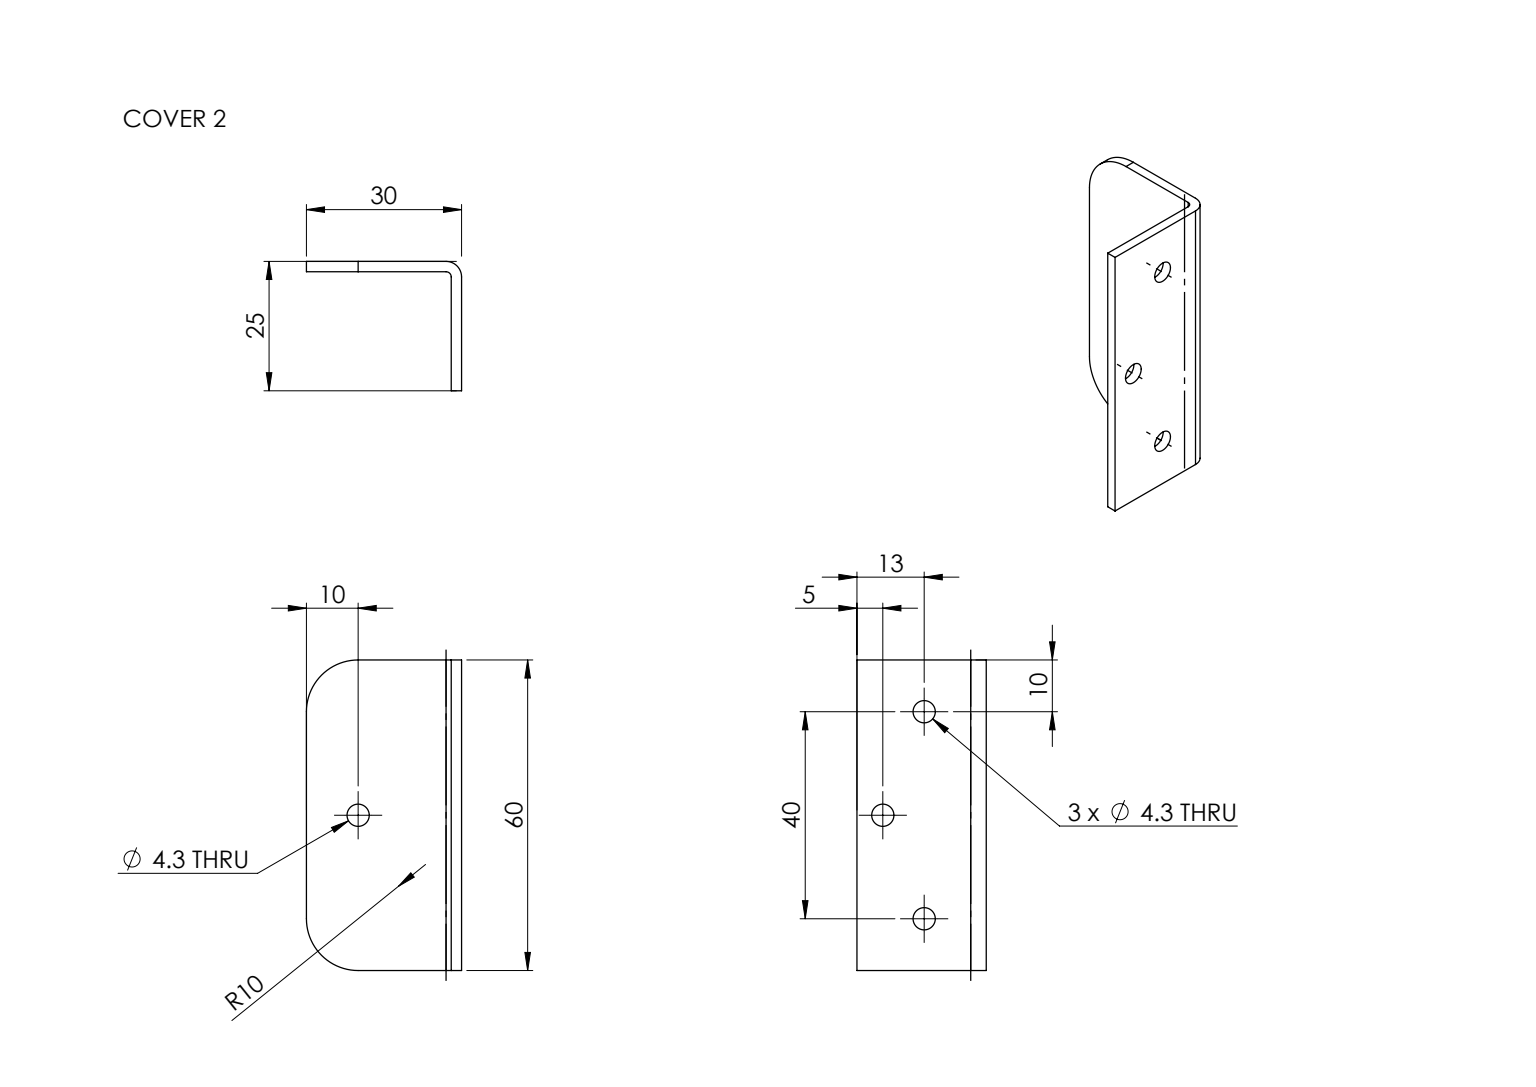
ISO-10303-21;
HEADER;
FILE_DESCRIPTION (('STEP AP214'),
    '1' );
FILE_NAME ('cover 2.step',
    '2026-10-03T20:08:58',
    ( '' ),
    ( '' ),
    'SwSTEP 2.0',
    'SolidWorks 2026',
    '' );
FILE_SCHEMA (( 'AUTOMOTIVE_DESIGN' ));
ENDSEC;

DATA;
#17=DIRECTION ( 'NONE',  ( 0.000000000000000000, 0.000000000000000000, 1.000000000000000000 ) ) ;
#30=LINE ( 'NONE', #10838, #312 ) ;
#47=VERTEX_POINT ( 'NONE', #5047 ) ;
#55=ORIENTED_EDGE ( 'NONE', *, *, #6653, .F. ) ;
#61=VECTOR ( 'NONE', #3554, 1000.000000000000000 ) ;
#80=CARTESIAN_POINT ( 'NONE',  ( -16.99999999999999289, 30.00000000000000000, 25.00000000000007105 ) ) ;
#104=FACE_OUTER_BOUND ( 'NONE', #9795, .T. ) ;
#120=EDGE_CURVE ( 'NONE', #10609, #7454, #4588, .T. ) ;
#131=DIRECTION ( 'NONE',  ( 0.000000000000000000, -1.177425296209236209E-30, -1.000000000000000000 ) ) ;
#140=CIRCLE ( 'NONE', #5087, 10.00000000000002309 ) ;
#209=COLOUR_RGB ( '', 0.66274510, 0.83137255, 0.94901961) ;
#213=EDGE_CURVE ( 'NONE', #4292, #815, #7867, .T. ) ;
#240=DIRECTION ( 'NONE',  ( -4.930380657631325535E-31, -1.000000000000000000, -1.177425296209239362E-30 ) ) ;
#259=CARTESIAN_POINT ( 'NONE',  ( -18.00000000000000355, 29.99999999999998224, 3.000000000000008438 ) ) ;
#261=CARTESIAN_POINT ( 'NONE',  ( -35.00000000000006395, 30.00000000000000000, 2.000000000000006661 ) ) ;
#263=CARTESIAN_POINT ( 'NONE',  ( -15.00000000000003375, 19.99999999999998934, 12.00000000000002842 ) ) ;
#279=CARTESIAN_POINT ( 'NONE',  ( -18.00000000000000355, 29.99999999999998224, 3.000000000000008438 ) ) ;
#280=( LENGTH_UNIT ( ) NAMED_UNIT ( * ) SI_UNIT ( .MILLI., .METRE. ) );
#302=VERTEX_POINT ( 'NONE', #12517 ) ;
#312=VECTOR ( 'NONE', #2087, 1000.000000000000000 ) ;
#352=CIRCLE ( 'NONE', #6535, 2.149999999999994138 ) ;
#364=VERTEX_POINT ( 'NONE', #10563 ) ;
#369=DIRECTION ( 'NONE',  ( 1.000000000000000000, 5.916456789157575403E-31, -1.577021341797098793E-16 ) ) ;
#455=CARTESIAN_POINT ( 'NONE',  ( -45.00000000000012079, -19.99999999999999645, 2.000000000000007994 ) ) ;
#471=DIRECTION ( 'NONE',  ( 0.000000000000000000, 0.000000000000000000, -1.000000000000000000 ) ) ;
#472=CARTESIAN_POINT ( 'NONE',  ( -17.00000000000000000, -30.00000000000000000, 3.000000000000030198 ) ) ;
#501=LINE ( 'NONE', #5270, #9745 ) ;
#507=EDGE_CURVE ( 'NONE', #8913, #7082, #5814, .T. ) ;
#509=VERTEX_POINT ( 'NONE', #8950 ) ;
#522=CARTESIAN_POINT ( 'NONE',  ( -18.00000000000002842, -30.00000000000000000, 4.336808689942017736E-16 ) ) ;
#538=CARTESIAN_POINT ( 'NONE',  ( -15.00000000000000000, 3.123110065765668157E-30, 22.15000000000006608 ) ) ;
#546=ORIENTED_EDGE ( 'NONE', *, *, #11077, .T. ) ;
#548=CARTESIAN_POINT ( 'NONE',  ( -15.00000000000003375, 19.99999999999998934, 12.00000000000002842 ) ) ;
#565=ORIENTED_EDGE ( 'NONE', *, *, #1103, .T. ) ;
#582=ORIENTED_EDGE ( 'NONE', *, *, #11922, .T. ) ;
#606=ADVANCED_FACE ( 'NONE', ( #5163 ), #9078, .F. ) ;
#609=DIRECTION ( 'NONE',  ( 1.000000000000000000, 5.916456789157575403E-31, -1.577021341797098793E-16 ) ) ;
#652=DIRECTION ( 'NONE',  ( -1.000000000000000000, -5.916456789157575403E-31, 1.577021341797098793E-16 ) ) ;
#681=LINE ( 'NONE', #4618, #8814 ) ;
#697=EDGE_LOOP ( 'NONE', ( #7888, #5340, #1354, #8282 ) ) ;
#703=CIRCLE ( 'NONE', #10980, 3.000000000000005773 ) ;
#708=EDGE_LOOP ( 'NONE', ( #5484, #4858 ) ) ;
#715=EDGE_CURVE ( 'NONE', #3334, #12136, #930, .T. ) ;
#724=PRODUCT ( 'cover 2', 'cover 2', '', ( #8914 ) ) ;
#734=DIRECTION ( 'NONE',  ( 1.000000000000000000, 5.916456789157575403E-31, -1.577021341797098793E-16 ) ) ;
#738=EDGE_LOOP ( 'NONE', ( #5945, #4675, #6555, #11845 ) ) ;
#749=VECTOR ( 'NONE', #6801, 1000.000000000000000 ) ;
#766=ADVANCED_FACE ( 'NONE', ( #4512, #5069, #893, #8688 ), #2728, .F. ) ;
#782=CARTESIAN_POINT ( 'NONE',  ( -35.00000000000006395, 19.99999999999999645, 2.000000000000006661 ) ) ;
#793=DIRECTION ( 'NONE',  ( 0.000000000000000000, 1.177425296209237785E-30, 1.000000000000000000 ) ) ;
#799=VECTOR ( 'NONE', #9430, 1000.000000000000000 ) ;
#808=AXIS2_PLACEMENT_3D ( 'NONE', #2794, #5790, #11854 ) ;
#813=DIRECTION ( 'NONE',  ( -1.000000000000000000, -5.916456789157575403E-31, 1.577021341797099039E-16 ) ) ;
#815=VERTEX_POINT ( 'NONE', #5661 ) ;
#822=ORIENTED_EDGE ( 'NONE', *, *, #9458, .T. ) ;
#834=CYLINDRICAL_SURFACE ( 'NONE', #10265, 2.149999999999999023 ) ;
#835=ORIENTED_EDGE ( 'NONE', *, *, #1795, .F. ) ;
#863=DIRECTION ( 'NONE',  ( -1.000000000000000000, -5.916456789157575403E-31, 1.577021341797098793E-16 ) ) ;
#884=AXIS2_PLACEMENT_3D ( 'NONE', #10014, #5142, #9121 ) ;
#893=FACE_BOUND ( 'NONE', #708, .T. ) ;
#926=DIRECTION ( 'NONE',  ( -1.000000000000000000, -5.916456789157575403E-31, 1.577021341797098793E-16 ) ) ;
#930=CIRCLE ( 'NONE', #7918, 10.00000000000002309 ) ;
#931=DIRECTION ( 'NONE',  ( 0.000000000000000000, 0.000000000000000000, -1.000000000000000000 ) ) ;
#954=LINE ( 'NONE', #3738, #5356 ) ;
#1019=CIRCLE ( 'NONE', #808, 2.149999999999994138 ) ;
#1060=DIRECTION ( 'NONE',  ( 1.000000000000000000, 5.916456789157575403E-31, -1.224646799147352714E-16 ) ) ;
#1071=ORIENTED_EDGE ( 'NONE', *, *, #6349, .F. ) ;
#1103=EDGE_CURVE ( 'NONE', #8313, #4963, #12522, .T. ) ;
#1114=EDGE_CURVE ( 'NONE', #11498, #6729, #11901, .T. ) ;
#1118=CYLINDRICAL_SURFACE ( 'NONE', #4514, 2.149999999999999023 ) ;
#1146=ORIENTED_EDGE ( 'NONE', *, *, #9111, .F. ) ;
#1156=DIRECTION ( 'NONE',  ( -4.930380657631325535E-31, -1.000000000000000000, -1.177425296209239362E-30 ) ) ;
#1166=DIRECTION ( 'NONE',  ( 0.000000000000000000, 0.000000000000000000, -1.000000000000000000 ) ) ;
#1176=DIRECTION ( 'NONE',  ( -4.930380657631325535E-31, -1.000000000000000000, -1.177425296209239362E-30 ) ) ;
#1179=AXIS2_PLACEMENT_3D ( 'NONE', #8679, #6694, #7716 ) ;
#1181=CARTESIAN_POINT ( 'NONE',  ( -18.00000000000001421, -30.00000000000001421, 3.000000000000008438 ) ) ;
#1199=ORIENTED_EDGE ( 'NONE', *, *, #5324, .F. ) ;
#1201=CARTESIAN_POINT ( 'NONE',  ( -18.00000000000002842, 30.00000000000000000, 4.336808689942017736E-16 ) ) ;
#1286=CARTESIAN_POINT ( 'NONE',  ( -15.00000000000000000, 2.465190328815661892E-29, 20.00000000000007461 ) ) ;
#1296=ADVANCED_FACE ( 'NONE', ( #7818 ), #3952, .T. ) ;
#1310=ORIENTED_EDGE ( 'NONE', *, *, #10574, .T. ) ;
#1318=ADVANCED_FACE ( 'NONE', ( #3131 ), #9024, .T. ) ;
#1354=ORIENTED_EDGE ( 'NONE', *, *, #5714, .F. ) ;
#1398=EDGE_CURVE ( 'NONE', #302, #815, #12426, .T. ) ;
#1402=DIRECTION ( 'NONE',  ( 1.000000000000000000, 5.916456789157575403E-31, -1.224646799147352714E-16 ) ) ;
#1452=CARTESIAN_POINT ( 'NONE',  ( -17.00000000000000000, 0.000000000000000000, 20.00000000000007461 ) ) ;
#1509=CARTESIAN_POINT ( 'NONE',  ( -45.00000000000001421, 19.99999999999999645, 3.443468848353431668E-15 ) ) ;
#1511=DIRECTION ( 'NONE',  ( -1.224646799147352714E-16, -1.177425296209236909E-30, -1.000000000000000000 ) ) ;
#1553=EDGE_CURVE ( 'NONE', #11498, #10609, #5066, .T. ) ;
#1561=CARTESIAN_POINT ( 'NONE',  ( -15.00000000000000711, -30.00000000000000000, 25.00000000000007105 ) ) ;
#1577=VERTEX_POINT ( 'NONE', #1907 ) ;
#1639=AXIS2_PLACEMENT_3D ( 'NONE', #5607, #12637, #7605 ) ;
#1662=CARTESIAN_POINT ( 'NONE',  ( -14.99999999999999289, 30.00000000000000000, 25.00000000000007105 ) ) ;
#1693=CARTESIAN_POINT ( 'NONE',  ( -15.00000000000000000, -20.00000000000000000, 14.15000000000002167 ) ) ;
#1702=CARTESIAN_POINT ( 'NONE',  ( -17.00000000000000000, 0.000000000000000000, 20.00000000000007461 ) ) ;
#1708=EDGE_CURVE ( 'NONE', #3334, #9611, #3336, .T. ) ;
#1734=VERTEX_POINT ( 'NONE', #11518 ) ;
#1766=DIRECTION ( 'NONE',  ( -1.000000000000000000, -5.916456789157575403E-31, 1.577021341797098793E-16 ) ) ;
#1779=( LENGTH_UNIT ( ) NAMED_UNIT ( * ) SI_UNIT ( .MILLI., .METRE. ) );
#1795=EDGE_CURVE ( 'NONE', #1734, #9663, #11530, .T. ) ;
#1850=AXIS2_PLACEMENT_3D ( 'NONE', #8562, #5785, #9765 ) ;
#1854=VECTOR ( 'NONE', #6775, 1000.000000000000000 ) ;
#1864=EDGE_CURVE ( 'NONE', #9310, #4937, #7061, .T. ) ;
#1886=ORIENTED_EDGE ( 'NONE', *, *, #6349, .T. ) ;
#1907=CARTESIAN_POINT ( 'NONE',  ( -15.00000000000003375, -30.00000000000000000, 3.000000000000029754 ) ) ;
#1922=ORIENTED_EDGE ( 'NONE', *, *, #7577, .F. ) ;
#1932=AXIS2_PLACEMENT_3D ( 'NONE', #2950, #3012, #4989 ) ;
#1936=CARTESIAN_POINT ( 'NONE',  ( -35.00000000000006395, -19.99999999999999645, 2.168404344971008868E-15 ) ) ;
#1941=LINE ( 'NONE', #6914, #4924 ) ;
#1958=DIRECTION ( 'NONE',  ( 0.000000000000000000, 1.177425296209236909E-30, 1.000000000000000000 ) ) ;
#1962=LINE ( 'NONE', #3904, #12124 ) ;
#1967=CARTESIAN_POINT ( 'NONE',  ( -35.00000000000006395, -2.157041537713704155E-29, 2.000000000000003553 ) ) ;
#1978=AXIS2_PLACEMENT_3D ( 'NONE', #1452, #926, #10645 ) ;
#2019=PRESENTATION_STYLE_ASSIGNMENT (( #6077 ) ) ;
#2087=DIRECTION ( 'NONE',  ( -2.465190328815656418E-32, 1.177425296209236734E-30, 1.000000000000000000 ) ) ;
#2088=AXIS2_PLACEMENT_3D ( 'NONE', #1286, #5281, #131 ) ;
#2104=AXIS2_PLACEMENT_3D ( 'NONE', #10365, #4392, #10559 ) ;
#2129=AXIS2_PLACEMENT_3D ( 'NONE', #3401, #12344, #3645 ) ;
#2143=( NAMED_UNIT ( * ) PLANE_ANGLE_UNIT ( ) SI_UNIT ( $, .RADIAN. ) );
#2145=ORIENTED_EDGE ( 'NONE', *, *, #10412, .T. ) ;
#2166=ORIENTED_EDGE ( 'NONE', *, *, #7676, .T. ) ;
#2167=CARTESIAN_POINT ( 'NONE',  ( -45.00000000000013500, 30.00000000000000000, 3.443468848353505426E-15 ) ) ;
#2207=CARTESIAN_POINT ( 'NONE',  ( -17.00000000000002842, 19.99999999999998579, 12.00000000000003730 ) ) ;
#2222=CARTESIAN_POINT ( 'NONE',  ( -18.00000000000002842, 30.00000000000000000, 2.000000000000004441 ) ) ;
#2233=DIRECTION ( 'NONE',  ( -1.000000000000000000, -5.916456789157575403E-31, 1.577021341797099039E-16 ) ) ;
#2244=EDGE_CURVE ( 'NONE', #11848, #1577, #6964, .T. ) ;
#2249=DIRECTION ( 'NONE',  ( 0.000000000000000000, 0.000000000000000000, -1.000000000000000000 ) ) ;
#2262=ORIENTED_EDGE ( 'NONE', *, *, #1795, .T. ) ;
#2285=MECHANICAL_DESIGN_GEOMETRIC_PRESENTATION_REPRESENTATION('',(#5766),#6810);
#2395=DIRECTION ( 'NONE',  ( -1.000000000000000000, 0.000000000000000000, 1.224646799147352714E-16 ) ) ;
#2408=CIRCLE ( 'NONE', #3443, 2.149999999999992362 ) ;
#2415=CARTESIAN_POINT ( 'NONE',  ( -17.00000000000002842, -20.00000000000000000, 9.850000000000047606 ) ) ;
#2421=ORIENTED_EDGE ( 'NONE', *, *, #8953, .T. ) ;
#2427=DIRECTION ( 'NONE',  ( -2.465190328815656418E-32, 1.177425296209236734E-30, 1.000000000000000000 ) ) ;
#2430=FACE_OUTER_BOUND ( 'NONE', #4109, .T. ) ;
#2442=CARTESIAN_POINT ( 'NONE',  ( -17.00000000000000000, 30.00000000000000000, 3.000000000000030198 ) ) ;
#2445=EDGE_LOOP ( 'NONE', ( #8731, #6641 ) ) ;
#2454=CARTESIAN_POINT ( 'NONE',  ( -16.99999999999999289, 30.00000000000000000, 25.00000000000007105 ) ) ;
#2494=DIRECTION ( 'NONE',  ( 0.000000000000000000, 0.000000000000000000, -1.000000000000000000 ) ) ;
#2500=FACE_OUTER_BOUND ( 'NONE', #3910, .T. ) ;
#2529=AXIS2_PLACEMENT_3D ( 'NONE', #11550, #2735, #9709 ) ;
#2583=PLANE ( 'NONE',  #11157 ) ;
#2592=CARTESIAN_POINT ( 'NONE',  ( -35.00000000000006395, -30.00000000000000000, 2.000000000000006661 ) ) ;
#2595=CARTESIAN_POINT ( 'NONE',  ( -15.00000000000000000, 30.00000000000000000, 3.000000000000029754 ) ) ;
#2597=EDGE_CURVE ( 'NONE', #4963, #9663, #954, .T. ) ;
#2635=FACE_BOUND ( 'NONE', #2445, .T. ) ;
#2648=FACE_BOUND ( 'NONE', #5059, .T. ) ;
#2695=VECTOR ( 'NONE', #1060, 1000.000000000000000 ) ;
#2697=EDGE_LOOP ( 'NONE', ( #5939, #9544, #4992, #8421 ) ) ;
#2710=DIRECTION ( 'NONE',  ( 1.000000000000000000, 5.916456789157576279E-31, 0.000000000000000000 ) ) ;
#2728=PLANE ( 'NONE',  #1850 ) ;
#2735=DIRECTION ( 'NONE',  ( -1.224646799147352714E-16, -1.177425296209236909E-30, -1.000000000000000000 ) ) ;
#2794=CARTESIAN_POINT ( 'NONE',  ( -17.00000000000002842, -20.00000000000000000, 12.00000000000003730 ) ) ;
#2825=APPLICATION_CONTEXT ( 'automotive_design' ) ;
#2839=CIRCLE ( 'NONE', #11249, 2.149999999999999023 ) ;
#2845=PRODUCT_DEFINITION_FORMATION_WITH_SPECIFIED_SOURCE ( 'ANY', '', #724, .NOT_KNOWN. ) ;
#2868=LINE ( 'NONE', #7803, #5698 ) ;
#2882=EDGE_CURVE ( 'NONE', #7500, #4292, #10406, .T. ) ;
#2883=LINE ( 'NONE', #5885, #749 ) ;
#2894=ORIENTED_EDGE ( 'NONE', *, *, #12398, .T. ) ;
#2912=ORIENTED_EDGE ( 'NONE', *, *, #2597, .T. ) ;
#2915=ORIENTED_EDGE ( 'NONE', *, *, #2244, .T. ) ;
#2949=AXIS2_PLACEMENT_3D ( 'NONE', #7795, #1156, #8946 ) ;
#2950=CARTESIAN_POINT ( 'NONE',  ( -35.00000000000006395, 19.99999999999999645, 2.000000000000007994 ) ) ;
#2964=ORIENTED_EDGE ( 'NONE', *, *, #1708, .F. ) ;
#3011=CARTESIAN_POINT ( 'NONE',  ( -17.00000000000002842, 19.99999999999998579, 12.00000000000003730 ) ) ;
#3012=DIRECTION ( 'NONE',  ( -2.465190328815656418E-32, 1.177425296209236734E-30, 1.000000000000000000 ) ) ;
#3015=AXIS2_PLACEMENT_3D ( 'NONE', #2222, #10051, #10116 ) ;
#3058=DIRECTION ( 'NONE',  ( -4.930380657631325535E-31, -1.000000000000000000, -1.177425296209239362E-30 ) ) ;
#3068=ORIENTED_EDGE ( 'NONE', *, *, #4877, .T. ) ;
#3074=ORIENTED_EDGE ( 'NONE', *, *, #11077, .F. ) ;
#3090=VECTOR ( 'NONE', #5249, 1000.000000000000000 ) ;
#3091=EDGE_LOOP ( 'NONE', ( #11028, #9675, #7446, #2915 ) ) ;
#3131=FACE_OUTER_BOUND ( 'NONE', #3091, .T. ) ;
#3143=ORIENTED_EDGE ( 'NONE', *, *, #5646, .T. ) ;
#3145=EDGE_CURVE ( 'NONE', #7082, #509, #5966, .T. ) ;
#3157=ORIENTED_EDGE ( 'NONE', *, *, #2882, .T. ) ;
#3175=ORIENTED_EDGE ( 'NONE', *, *, #12697, .T. ) ;
#3183=EDGE_CURVE ( 'NONE', #8913, #47, #6026, .T. ) ;
#3198=CARTESIAN_POINT ( 'NONE',  ( -32.85000000000007248, -2.147580246367739864E-29, 1.905105283154350624E-15 ) ) ;
#3199=ORIENTED_EDGE ( 'NONE', *, *, #5959, .T. ) ;
#3200=VECTOR ( 'NONE', #11397, 1000.000000000000000 ) ;
#3206=( NAMED_UNIT ( * ) SI_UNIT ( $, .STERADIAN. ) SOLID_ANGLE_UNIT ( ) );
#3223=AXIS2_PLACEMENT_3D ( 'NONE', #1181, #9032, #931 ) ;
#3242=VERTEX_POINT ( 'NONE', #6339 ) ;
#3244=ORIENTED_EDGE ( 'NONE', *, *, #8545, .T. ) ;
#3252=FACE_BOUND ( 'NONE', #3650, .T. ) ;
#3267=CARTESIAN_POINT ( 'NONE',  ( -18.00000000000001421, 29.99999999999999289, 2.000000000000004885 ) ) ;
#3283=VECTOR ( 'NONE', #813, 1000.000000000000000 ) ;
#3334=VERTEX_POINT ( 'NONE', #1509 ) ;
#3336=LINE ( 'NONE', #2167, #3090 ) ;
#3338=FACE_OUTER_BOUND ( 'NONE', #738, .T. ) ;
#3362=ADVANCED_FACE ( 'NONE', ( #7378 ), #10319, .F. ) ;
#3401=CARTESIAN_POINT ( 'NONE',  ( -17.00000000000002842, -20.00000000000000000, 12.00000000000003730 ) ) ;
#3405=ORIENTED_EDGE ( 'NONE', *, *, #507, .F. ) ;
#3407=ADVANCED_FACE ( 'NONE', ( #3584 ), #5311, .F. ) ;
#3408=PLANE ( 'NONE',  #3510 ) ;
#3439=ORIENTED_EDGE ( 'NONE', *, *, #10966, .T. ) ;
#3443=AXIS2_PLACEMENT_3D ( 'NONE', #1702, #1766, #793 ) ;
#3510=AXIS2_PLACEMENT_3D ( 'NONE', #5318, #12165, #4355 ) ;
#3519=STYLED_ITEM ( 'NONE', ( #11091 ), #9701 ) ;
#3546=AXIS2_PLACEMENT_3D ( 'NONE', #259, #4191, #8110 ) ;
#3554=DIRECTION ( 'NONE',  ( 1.000000000000000000, 5.916456789157575403E-31, -1.224646799147352714E-16 ) ) ;
#3584=FACE_OUTER_BOUND ( 'NONE', #11187, .T. ) ;
#3645=DIRECTION ( 'NONE',  ( 0.000000000000000000, 0.000000000000000000, 1.000000000000000000 ) ) ;
#3650=EDGE_LOOP ( 'NONE', ( #10523, #4157 ) ) ;
#3653=EDGE_LOOP ( 'NONE', ( #11585, #10453, #10007, #3765, #5718, #6710 ) ) ;
#3694=VECTOR ( 'NONE', #11699, 1000.000000000000000 ) ;
#3699=CARTESIAN_POINT ( 'NONE',  ( -18.00000000000001421, -30.00000000000001421, 3.000000000000008438 ) ) ;
#3734=DIRECTION ( 'NONE',  ( 5.916456789157575403E-31, -1.000000000000000000, -1.177425296209239362E-30 ) ) ;
#3738=CARTESIAN_POINT ( 'NONE',  ( -32.85000000000006537, -2.029837716746816226E-29, 2.000000000000002220 ) ) ;
#3765=ORIENTED_EDGE ( 'NONE', *, *, #12715, .T. ) ;
#3773=EDGE_CURVE ( 'NONE', #6729, #7454, #11229, .T. ) ;
#3795=DIRECTION ( 'NONE',  ( -2.465190328815656418E-32, 1.177425296209236734E-30, 1.000000000000000000 ) ) ;
#3904=CARTESIAN_POINT ( 'NONE',  ( -45.00000000000001421, 19.99999999999999645, 3.469446951953614189E-15 ) ) ;
#3910=EDGE_LOOP ( 'NONE', ( #9964, #4431, #3439, #2166 ) ) ;
#3940=DIRECTION ( 'NONE',  ( -4.930380657631325535E-31, -1.000000000000000000, -1.177425296209239362E-30 ) ) ;
#3952=PLANE ( 'NONE',  #5930 ) ;
#3956=VECTOR ( 'NONE', #6375, 1000.000000000000000 ) ;
#3984=DIRECTION ( 'NONE',  ( -2.465190328815656418E-32, 1.177425296209236734E-30, 1.000000000000000000 ) ) ;
#4014=DIRECTION ( 'NONE',  ( 1.000000000000000000, 5.916456789157575403E-31, 2.465190328815656418E-32 ) ) ;
#4067=SURFACE_SIDE_STYLE ('',( #8119 ) ) ;
#4109=EDGE_LOOP ( 'NONE', ( #6272, #6518, #11240, #8208 ) ) ;
#4134=FILL_AREA_STYLE ('',( #7708 ) ) ;
#4141=CARTESIAN_POINT ( 'NONE',  ( -18.00000000000000355, 29.99999999999998224, 3.000000000000008438 ) ) ;
#4157=ORIENTED_EDGE ( 'NONE', *, *, #1103, .F. ) ;
#4191=DIRECTION ( 'NONE',  ( -4.930380657631325535E-31, -1.000000000000000000, -1.177425296209239362E-30 ) ) ;
#4213=ORIENTED_EDGE ( 'NONE', *, *, #7256, .T. ) ;
#4231=ORIENTED_EDGE ( 'NONE', *, *, #1553, .T. ) ;
#4250=VERTEX_POINT ( 'NONE', #1662 ) ;
#4262=AXIS2_PLACEMENT_3D ( 'NONE', #5297, #9980, #7244 ) ;
#4282=DIRECTION ( 'NONE',  ( -1.000000000000000000, -5.916456789157575403E-31, 1.577021341797099039E-16 ) ) ;
#4292=VERTEX_POINT ( 'NONE', #10660 ) ;
#4312=CARTESIAN_POINT ( 'NONE',  ( -17.00000000000000000, 30.00000000000000000, 3.000000000000030198 ) ) ;
#4319=ADVANCED_FACE ( 'NONE', ( #104 ), #6821, .T. ) ;
#4331=CARTESIAN_POINT ( 'NONE',  ( -17.00000000000002842, -20.00000000000000000, 9.850000000000036948 ) ) ;
#4349=CARTESIAN_POINT ( 'NONE',  ( -35.00000000000006395, -19.99999999999999645, 3.000000000000008438 ) ) ;
#4355=DIRECTION ( 'NONE',  ( -1.577021341797098546E-16, -1.177425296209237084E-30, -1.000000000000000000 ) ) ;
#4392=DIRECTION ( 'NONE',  ( -1.000000000000000000, -5.916456789157575403E-31, 1.577021341797098793E-16 ) ) ;
#4431=ORIENTED_EDGE ( 'NONE', *, *, #2244, .F. ) ;
#4469=VECTOR ( 'NONE', #8952, 1000.000000000000000 ) ;
#4512=FACE_OUTER_BOUND ( 'NONE', #697, .T. ) ;
#4514=AXIS2_PLACEMENT_3D ( 'NONE', #8971, #8004, #1958 ) ;
#4570=LINE ( 'NONE', #8548, #3200 ) ;
#4588=CIRCLE ( 'NONE', #10542, 2.149999999999994138 ) ;
#4607=ORIENTED_EDGE ( 'NONE', *, *, #7208, .F. ) ;
#4618=CARTESIAN_POINT ( 'NONE',  ( -15.00000000000000000, 30.00000000000000000, 3.000000000000029754 ) ) ;
#4675=ORIENTED_EDGE ( 'NONE', *, *, #7256, .F. ) ;
#4706=LINE ( 'NONE', #12578, #6378 ) ;
#4734=DIRECTION ( 'NONE',  ( 1.000000000000000000, 5.916456789157576279E-31, 0.000000000000000000 ) ) ;
#4740=ADVANCED_FACE ( 'NONE', ( #2430 ), #6342, .F. ) ;
#4746=ORIENTED_EDGE ( 'NONE', *, *, #5952, .F. ) ;
#4788=UNCERTAINTY_MEASURE_WITH_UNIT (LENGTH_MEASURE( 1.000000000000000082E-05 ), #10955, 'distance_accuracy_value', 'NONE');
#4796=CIRCLE ( 'NONE', #884, 10.00000000000002309 ) ;
#4804=AXIS2_PLACEMENT_3D ( 'NONE', #12219, #2427, #4854 ) ;
#4854=DIRECTION ( 'NONE',  ( 1.000000000000000000, 5.916456789157576279E-31, 0.000000000000000000 ) ) ;
#4858=ORIENTED_EDGE ( 'NONE', *, *, #11792, .F. ) ;
#4876=AXIS2_PLACEMENT_3D ( 'NONE', #4349, #9229, #8276 ) ;
#4877=EDGE_CURVE ( 'NONE', #3242, #9347, #2883, .T. ) ;
#4924=VECTOR ( 'NONE', #6972, 1000.000000000000000 ) ;
#4937=VERTEX_POINT ( 'NONE', #6073 ) ;
#4963=VERTEX_POINT ( 'NONE', #3198 ) ;
#4989=DIRECTION ( 'NONE',  ( 1.000000000000000000, 0.000000000000000000, 0.000000000000000000 ) ) ;
#4992=ORIENTED_EDGE ( 'NONE', *, *, #11792, .T. ) ;
#5043=( NAMED_UNIT ( * ) SI_UNIT ( $, .STERADIAN. ) SOLID_ANGLE_UNIT ( ) );
#5047=CARTESIAN_POINT ( 'NONE',  ( -17.00000000000000000, 2.531464386849852200E-30, 22.15000000000006608 ) ) ;
#5059=EDGE_LOOP ( 'NONE', ( #3405, #12376 ) ) ;
#5061=ORIENTED_EDGE ( 'NONE', *, *, #10966, .F. ) ;
#5066=LINE ( 'NONE', #11642, #3694 ) ;
#5069=FACE_BOUND ( 'NONE', #12624, .T. ) ;
#5087=AXIS2_PLACEMENT_3D ( 'NONE', #1936, #12520, #7616 ) ;
#5116=( NAMED_UNIT ( * ) PLANE_ANGLE_UNIT ( ) SI_UNIT ( $, .RADIAN. ) );
#5123=ORIENTED_EDGE ( 'NONE', *, *, #11983, .F. ) ;
#5128=CIRCLE ( 'NONE', #11295, 2.149999999999999023 ) ;
#5141=AXIS2_PLACEMENT_3D ( 'NONE', #1967, #10535, #2710 ) ;
#5142=DIRECTION ( 'NONE',  ( 1.224646799147352714E-16, 1.177425296209236909E-30, 1.000000000000000000 ) ) ;
#5163=FACE_OUTER_BOUND ( 'NONE', #8488, .T. ) ;
#5217=EDGE_LOOP ( 'NONE', ( #11701, #3199, #3068, #3244, #2421, #7025, #1199, #6196 ) ) ;
#5249=DIRECTION ( 'NONE',  ( -4.930380657631325535E-31, -1.000000000000000000, -1.177425296209239362E-30 ) ) ;
#5250=CARTESIAN_POINT ( 'NONE',  ( -17.00000000000000000, 2.531464386849858155E-30, 22.15000000000007319 ) ) ;
#5270=CARTESIAN_POINT ( 'NONE',  ( -18.00000000000002842, 30.00000000000000000, 2.000000000000004441 ) ) ;
#5276=ORIENTED_EDGE ( 'NONE', *, *, #3773, .T. ) ;
#5281=DIRECTION ( 'NONE',  ( 1.000000000000000000, 5.916456789157575403E-31, -1.577021341797098793E-16 ) ) ;
#5297=CARTESIAN_POINT ( 'NONE',  ( -17.00000000000002842, -20.00000000000000000, 12.00000000000003730 ) ) ;
#5301=EDGE_CURVE ( 'NONE', #3242, #9611, #140, .T. ) ;
#5311=CYLINDRICAL_SURFACE ( 'NONE', #4804, 2.149999999999999023 ) ;
#5318=CARTESIAN_POINT ( 'NONE',  ( -15.00000000000000000, 30.00000000000000000, 3.000000000000029754 ) ) ;
#5324=EDGE_CURVE ( 'NONE', #10180, #8458, #11806, .T. ) ;
#5340=ORIENTED_EDGE ( 'NONE', *, *, #12250, .F. ) ;
#5356=VECTOR ( 'NONE', #3984, 1000.000000000000000 ) ;
#5359=CARTESIAN_POINT ( 'NONE',  ( -17.00000000000002842, 19.99999999999998579, 12.00000000000003730 ) ) ;
#5397=DIRECTION ( 'NONE',  ( -2.465190328815656418E-32, 1.177425296209236734E-30, 1.000000000000000000 ) ) ;
#5399=CARTESIAN_POINT ( 'NONE',  ( -16.99999999999999289, -30.00000000000000000, 25.00000000000007105 ) ) ;
#5404=CARTESIAN_POINT ( 'NONE',  ( -35.00000000000006395, 30.00000000000000000, 2.218822049206179977E-15 ) ) ;
#5423=ORIENTED_EDGE ( 'NONE', *, *, #5431, .T. ) ;
#5431=EDGE_CURVE ( 'NONE', #815, #4292, #352, .T. ) ;
#5444=DIRECTION ( 'NONE',  ( 0.000000000000000000, 0.000000000000000000, -1.000000000000000000 ) ) ;
#5480=AXIS2_PLACEMENT_3D ( 'NONE', #10079, #369, #2249 ) ;
#5484=ORIENTED_EDGE ( 'NONE', *, *, #5909, .F. ) ;
#5526=EDGE_LOOP ( 'NONE', ( #11382, #5843, #1886, #12256 ) ) ;
#5531=CARTESIAN_POINT ( 'NONE',  ( -32.85000000000006537, -2.029837716746816226E-29, 2.000000000000003553 ) ) ;
#5535=DIRECTION ( 'NONE',  ( -1.000000000000000000, -5.916456789157575403E-31, -2.465190328815656418E-32 ) ) ;
#5583=ORIENTED_EDGE ( 'NONE', *, *, #9111, .T. ) ;
#5607=CARTESIAN_POINT ( 'NONE',  ( -15.00000000000000000, 2.465190328815661892E-29, 20.00000000000007461 ) ) ;
#5609=AXIS2_PLACEMENT_3D ( 'NONE', #5359, #652, #6592 ) ;
#5646=EDGE_CURVE ( 'NONE', #6729, #11498, #9769, .T. ) ;
#5661=CARTESIAN_POINT ( 'NONE',  ( -17.00000000000002842, 19.99999999999998579, 14.15000000000003055 ) ) ;
#5692=CARTESIAN_POINT ( 'NONE',  ( -35.00000000000006395, -2.157041537713704155E-29, 2.000000000000003553 ) ) ;
#5698=VECTOR ( 'NONE', #5927, 1000.000000000000000 ) ;
#5707=CARTESIAN_POINT ( 'NONE',  ( 0.000000000000000000, 0.000000000000000000, 0.000000000000000000 ) ) ;
#5713=ORIENTED_EDGE ( 'NONE', *, *, #8690, .F. ) ;
#5714=EDGE_CURVE ( 'NONE', #12227, #11665, #7395, .T. ) ;
#5718=ORIENTED_EDGE ( 'NONE', *, *, #1864, .T. ) ;
#5719=LINE ( 'NONE', #9630, #10320 ) ;
#5747=AXIS2_PLACEMENT_3D ( 'NONE', #3699, #11559, #11023 ) ;
#5750=AXIS2_PLACEMENT_3D ( 'NONE', #6673, #1511, #10584 ) ;
#5765=( GEOMETRIC_REPRESENTATION_CONTEXT ( 3 ) GLOBAL_UNCERTAINTY_ASSIGNED_CONTEXT ( ( #11494 ) ) GLOBAL_UNIT_ASSIGNED_CONTEXT ( ( #1779, #12482, #5043 ) ) REPRESENTATION_CONTEXT ( 'NONE', 'WORKASPACE' ) );
#5766=STYLED_ITEM ( 'NONE', ( #2019 ), #10029 ) ;
#5785=DIRECTION ( 'NONE',  ( 1.000000000000000000, 5.916456789157575403E-31, -1.577021341797098546E-16 ) ) ;
#5790=DIRECTION ( 'NONE',  ( -1.000000000000000000, -5.916456789157575403E-31, 1.577021341797098793E-16 ) ) ;
#5798=CIRCLE ( 'NONE', #2529, 2.149999999999999023 ) ;
#5805=CARTESIAN_POINT ( 'NONE',  ( -17.00000000000002842, 19.99999999999998579, 12.00000000000003730 ) ) ;
#5809=ADVANCED_FACE ( 'NONE', ( #3338 ), #10186, .T. ) ;
#5814=CIRCLE ( 'NONE', #2088, 2.149999999999999023 ) ;
#5828=ORIENTED_EDGE ( 'NONE', *, *, #1553, .F. ) ;
#5843=ORIENTED_EDGE ( 'NONE', *, *, #7676, .F. ) ;
#5885=CARTESIAN_POINT ( 'NONE',  ( -18.00000000000002842, -30.00000000000000000, 1.369224906555730040E-16 ) ) ;
#5909=EDGE_CURVE ( 'NONE', #47, #509, #2408, .T. ) ;
#5913=ORIENTED_EDGE ( 'NONE', *, *, #120, .F. ) ;
#5923=EDGE_CURVE ( 'NONE', #9663, #1734, #6930, .T. ) ;
#5927=DIRECTION ( 'NONE',  ( -1.000000000000000000, -5.916456789157575403E-31, -2.465190328815656418E-32 ) ) ;
#5930=AXIS2_PLACEMENT_3D ( 'NONE', #11816, #10832, #4014 ) ;
#5939=ORIENTED_EDGE ( 'NONE', *, *, #507, .T. ) ;
#5945=ORIENTED_EDGE ( 'NONE', *, *, #12715, .F. ) ;
#5946=DIRECTION ( 'NONE',  ( 0.000000000000000000, 0.000000000000000000, 1.000000000000000000 ) ) ;
#5952=EDGE_CURVE ( 'NONE', #302, #7500, #2839, .T. ) ;
#5959=EDGE_CURVE ( 'NONE', #9310, #3242, #6413, .T. ) ;
#5963=AXIS2_PLACEMENT_3D ( 'NONE', #8893, #3058, #6973 ) ;
#5966=LINE ( 'NONE', #7257, #9914 ) ;
#6018=ORIENTED_EDGE ( 'NONE', *, *, #120, .T. ) ;
#6026=LINE ( 'NONE', #5250, #12418 ) ;
#6062=DIRECTION ( 'NONE',  ( 1.000000000000000000, 5.916456789157575403E-31, -1.577021341797098793E-16 ) ) ;
#6073=CARTESIAN_POINT ( 'NONE',  ( -18.00000000000001421, -30.00000000000000711, 2.000000000000004885 ) ) ;
#6075=FACE_BOUND ( 'NONE', #6886, .T. ) ;
#6077=SURFACE_STYLE_USAGE ( .BOTH. , #8065 ) ;
#6086=ADVANCED_FACE ( 'NONE', ( #8261 ), #11162, .F. ) ;
#6102=LINE ( 'NONE', #1201, #11999 ) ;
#6112=VECTOR ( 'NONE', #8579, 1000.000000000000000 ) ;
#6125=DIRECTION ( 'NONE',  ( -1.000000000000000000, -5.916456789157575403E-31, 1.577021341797098793E-16 ) ) ;
#6133=CARTESIAN_POINT ( 'NONE',  ( -17.00000000000002842, -20.00000000000000000, 12.00000000000003730 ) ) ;
#6135=AXIS2_PLACEMENT_3D ( 'NONE', #4141, #1176, #7046 ) ;
#6196=ORIENTED_EDGE ( 'NONE', *, *, #10412, .F. ) ;
#6239=EDGE_CURVE ( 'NONE', #8666, #8458, #10305, .T. ) ;
#6272=ORIENTED_EDGE ( 'NONE', *, *, #3145, .F. ) ;
#6290=ORIENTED_EDGE ( 'NONE', *, *, #715, .T. ) ;
#6316=DIRECTION ( 'NONE',  ( -1.000000000000000000, -5.916456789157575403E-31, 1.224646799147352714E-16 ) ) ;
#6339=CARTESIAN_POINT ( 'NONE',  ( -35.00000000000006395, -30.00000000000000000, 2.218822049206081369E-15 ) ) ;
#6342=CYLINDRICAL_SURFACE ( 'NONE', #1978, 2.149999999999999023 ) ;
#6349=EDGE_CURVE ( 'NONE', #4250, #11665, #2868, .T. ) ;
#6375=DIRECTION ( 'NONE',  ( -4.930380657631325535E-31, -1.000000000000000000, -1.177425296209239362E-30 ) ) ;
#6378=VECTOR ( 'NONE', #6519, 1000.000000000000000 ) ;
#6413=LINE ( 'NONE', #12662, #6525 ) ;
#6428=DIRECTION ( 'NONE',  ( 1.000000000000000000, 0.000000000000000000, 0.000000000000000000 ) ) ;
#6430=DIRECTION ( 'NONE',  ( 1.577021341797099039E-16, 1.177425296209237084E-30, 1.000000000000000000 ) ) ;
#6431=ORIENTED_EDGE ( 'NONE', *, *, #715, .F. ) ;
#6443=ORIENTED_EDGE ( 'NONE', *, *, #1398, .F. ) ;
#6507=ORIENTED_EDGE ( 'NONE', *, *, #5923, .F. ) ;
#6518=ORIENTED_EDGE ( 'NONE', *, *, #10714, .T. ) ;
#6519=DIRECTION ( 'NONE',  ( -4.930380657631325535E-31, -1.000000000000000000, -1.177425296209239362E-30 ) ) ;
#6525=VECTOR ( 'NONE', #7757, 1000.000000000000000 ) ;
#6529=EDGE_CURVE ( 'NONE', #7823, #8669, #501, .T. ) ;
#6533=DIRECTION ( 'NONE',  ( -1.000000000000000000, 0.000000000000000000, 1.301042606982602363E-16 ) ) ;
#6535=AXIS2_PLACEMENT_3D ( 'NONE', #2207, #6125, #10034 ) ;
#6538=FACE_OUTER_BOUND ( 'NONE', #5217, .T. ) ;
#6555=ORIENTED_EDGE ( 'NONE', *, *, #5301, .F. ) ;
#6560=ORIENTED_EDGE ( 'NONE', *, *, #6612, .T. ) ;
#6569=ORIENTED_EDGE ( 'NONE', *, *, #1398, .T. ) ;
#6592=DIRECTION ( 'NONE',  ( 0.000000000000000000, 0.000000000000000000, 1.000000000000000000 ) ) ;
#6612=EDGE_CURVE ( 'NONE', #12136, #7823, #11267, .T. ) ;
#6641=ORIENTED_EDGE ( 'NONE', *, *, #5646, .F. ) ;
#6653=EDGE_CURVE ( 'NONE', #12092, #7976, #4570, .T. ) ;
#6673=CARTESIAN_POINT ( 'NONE',  ( -35.00000000000006395, -2.157041537713704155E-29, 2.168404344971033323E-15 ) ) ;
#6694=DIRECTION ( 'NONE',  ( -1.000000000000000000, -5.916456789157575403E-31, -2.465190328815656418E-32 ) ) ;
#6710=ORIENTED_EDGE ( 'NONE', *, *, #10574, .F. ) ;
#6729=VERTEX_POINT ( 'NONE', #11587 ) ;
#6775=DIRECTION ( 'NONE',  ( -4.930380657631325535E-31, -1.000000000000000000, -1.177425296209239362E-30 ) ) ;
#6776=AXIS2_PLACEMENT_3D ( 'NONE', #11279, #11996, #6316 ) ;
#6784=CARTESIAN_POINT ( 'NONE',  ( -14.99999999999999289, 30.00000000000000000, 25.00000000000007105 ) ) ;
#6801=DIRECTION ( 'NONE',  ( 1.000000000000000000, 5.916456789157575403E-31, -1.224646799147352714E-16 ) ) ;
#6803=CARTESIAN_POINT ( 'NONE',  ( -17.00000000000000000, 30.00000000000000000, 3.000000000000030198 ) ) ;
#6809=EDGE_LOOP ( 'NONE', ( #2964, #6290, #11253, #3175, #8753, #10302 ) ) ;
#6810=( GEOMETRIC_REPRESENTATION_CONTEXT ( 3 ) GLOBAL_UNCERTAINTY_ASSIGNED_CONTEXT ( ( #8653 ) ) GLOBAL_UNIT_ASSIGNED_CONTEXT ( ( #280, #5116, #3206 ) ) REPRESENTATION_CONTEXT ( 'NONE', 'WORKASPACE' ) );
#6812=SURFACE_STYLE_USAGE ( .BOTH. , #4067 ) ;
#6821=PLANE ( 'NONE',  #1179 ) ;
#6874=SHAPE_DEFINITION_REPRESENTATION ( #8540, #11514 ) ;
#6886=EDGE_LOOP ( 'NONE', ( #6507, #835 ) ) ;
#6914=CARTESIAN_POINT ( 'NONE',  ( -15.00000000000003375, -30.00000000000000000, 3.000000000000029754 ) ) ;
#6927=DIRECTION ( 'NONE',  ( -4.930380657631325535E-31, -1.000000000000000000, -1.177425296209239362E-30 ) ) ;
#6930=CIRCLE ( 'NONE', #9576, 2.149999999999999023 ) ;
#6964=LINE ( 'NONE', #11923, #1854 ) ;
#6972=DIRECTION ( 'NONE',  ( 1.577021341797099039E-16, 1.177425296209237084E-30, 1.000000000000000000 ) ) ;
#6973=DIRECTION ( 'NONE',  ( 1.000000000000000000, 0.000000000000000000, -6.375108774214761023E-14 ) ) ;
#7025=ORIENTED_EDGE ( 'NONE', *, *, #6239, .T. ) ;
#7046=DIRECTION ( 'NONE',  ( 0.000000000000000000, 0.000000000000000000, -1.000000000000000000 ) ) ;
#7052=FILL_AREA_STYLE ('',( #11760 ) ) ;
#7061=LINE ( 'NONE', #10913, #2695 ) ;
#7082=VERTEX_POINT ( 'NONE', #12474 ) ;
#7106=ORIENTED_EDGE ( 'NONE', *, *, #213, .T. ) ;
#7117=VECTOR ( 'NONE', #3940, 1000.000000000000000 ) ;
#7118=ORIENTED_EDGE ( 'NONE', *, *, #2882, .F. ) ;
#7164=CARTESIAN_POINT ( 'NONE',  ( -17.00000000000000000, -30.00000000000000000, 3.000000000000030198 ) ) ;
#7208=EDGE_CURVE ( 'NONE', #12227, #10180, #12728, .T. ) ;
#7242=ADVANCED_FACE ( 'NONE', ( #8844 ), #7878, .F. ) ;
#7244=DIRECTION ( 'NONE',  ( 0.000000000000000000, 0.000000000000000000, 1.000000000000000000 ) ) ;
#7256=EDGE_CURVE ( 'NONE', #9611, #7976, #30, .T. ) ;
#7257=CARTESIAN_POINT ( 'NONE',  ( -17.00000000000000000, 2.632990618166788035E-16, 17.85000000000007248 ) ) ;
#7274=EDGE_LOOP ( 'NONE', ( #1922, #9378, #6431, #3074 ) ) ;
#7307=FACE_OUTER_BOUND ( 'NONE', #3653, .T. ) ;
#7340=ADVANCED_FACE ( 'NONE', ( #6075, #7307 ), #9281, .F. ) ;
#7346=ORIENTED_EDGE ( 'NONE', *, *, #5952, .T. ) ;
#7355=PLANE ( 'NONE',  #6776 ) ;
#7378=FACE_OUTER_BOUND ( 'NONE', #9057, .T. ) ;
#7392=DIRECTION ( 'NONE',  ( 0.000000000000000000, 0.000000000000000000, 1.000000000000000000 ) ) ;
#7395=LINE ( 'NONE', #2442, #12692 ) ;
#7407=AXIS2_PLACEMENT_3D ( 'NONE', #9411, #609, #5444 ) ;
#7446=ORIENTED_EDGE ( 'NONE', *, *, #8690, .T. ) ;
#7454=VERTEX_POINT ( 'NONE', #2415 ) ;
#7457=CARTESIAN_POINT ( 'NONE',  ( -17.00000000000002842, 19.99999999999998579, 14.15000000000003588 ) ) ;
#7500=VERTEX_POINT ( 'NONE', #8389 ) ;
#7510=AXIS2_PLACEMENT_3D ( 'NONE', #3011, #863, #5946 ) ;
#7577=EDGE_CURVE ( 'NONE', #7823, #12092, #12466, .T. ) ;
#7605=DIRECTION ( 'NONE',  ( 0.000000000000000000, -1.177425296209236209E-30, -1.000000000000000000 ) ) ;
#7616=DIRECTION ( 'NONE',  ( -1.000000000000000000, 0.000000000000000000, 1.224646799147352714E-16 ) ) ;
#7676=EDGE_CURVE ( 'NONE', #4250, #8666, #10633, .T. ) ;
#7703=DIRECTION ( 'NONE',  ( 2.465190328815656418E-32, -1.177425296209236734E-30, -1.000000000000000000 ) ) ;
#7704=EDGE_LOOP ( 'NONE', ( #7346, #3157, #7106, #6443 ) ) ;
#7708=FILL_AREA_STYLE_COLOUR ( '', #209 ) ;
#7716=DIRECTION ( 'NONE',  ( -2.465190328815656418E-32, 1.177425296209236734E-30, 1.000000000000000000 ) ) ;
#7757=DIRECTION ( 'NONE',  ( 2.465190328815656418E-32, -1.177425296209236734E-30, -1.000000000000000000 ) ) ;
#7795=CARTESIAN_POINT ( 'NONE',  ( -18.00000000000000355, 29.99999999999998224, 3.000000000000008438 ) ) ;
#7803=CARTESIAN_POINT ( 'NONE',  ( -14.99999999999999289, 30.00000000000000000, 25.00000000000007105 ) ) ;
#7818=FACE_OUTER_BOUND ( 'NONE', #5526, .T. ) ;
#7823=VERTEX_POINT ( 'NONE', #261 ) ;
#7825=FACE_OUTER_BOUND ( 'NONE', #7274, .T. ) ;
#7867=CIRCLE ( 'NONE', #5609, 2.149999999999994138 ) ;
#7878=CYLINDRICAL_SURFACE ( 'NONE', #7510, 2.149999999999999023 ) ;
#7888=ORIENTED_EDGE ( 'NONE', *, *, #5324, .T. ) ;
#7918=AXIS2_PLACEMENT_3D ( 'NONE', #8372, #12248, #2395 ) ;
#7976=VERTEX_POINT ( 'NONE', #455 ) ;
#8004=DIRECTION ( 'NONE',  ( -1.000000000000000000, -5.916456789157575403E-31, 1.577021341797098793E-16 ) ) ;
#8046=CIRCLE ( 'NONE', #2104, 2.149999999999992362 ) ;
#8065=SURFACE_SIDE_STYLE ('',( #10774 ) ) ;
#8105=LINE ( 'NONE', #2454, #3956 ) ;
#8110=DIRECTION ( 'NONE',  ( 0.000000000000000000, 0.000000000000000000, -1.000000000000000000 ) ) ;
#8119=SURFACE_STYLE_FILL_AREA ( #4134 ) ;
#8208=ORIENTED_EDGE ( 'NONE', *, *, #5909, .T. ) ;
#8260=DIRECTION ( 'NONE',  ( -1.000000000000000000, -5.916456789157575403E-31, 1.577021341797099039E-16 ) ) ;
#8261=FACE_OUTER_BOUND ( 'NONE', #12309, .T. ) ;
#8276=DIRECTION ( 'NONE',  ( -1.000000000000000000, 0.000000000000000000, 0.000000000000000000 ) ) ;
#8282=ORIENTED_EDGE ( 'NONE', *, *, #7208, .T. ) ;
#8291=CARTESIAN_POINT ( 'NONE',  ( -17.00000000000002842, 19.99999999999998579, 9.850000000000036948 ) ) ;
#8313=VERTEX_POINT ( 'NONE', #9194 ) ;
#8372=CARTESIAN_POINT ( 'NONE',  ( -35.00000000000006395, 19.99999999999999645, 2.168404344971058172E-15 ) ) ;
#8389=CARTESIAN_POINT ( 'NONE',  ( -15.00000000000003375, 19.99999999999998579, 9.850000000000033396 ) ) ;
#8408=ORIENTED_EDGE ( 'NONE', *, *, #12398, .F. ) ;
#8421=ORIENTED_EDGE ( 'NONE', *, *, #3183, .F. ) ;
#8458=VERTEX_POINT ( 'NONE', #5399 ) ;
#8488=EDGE_LOOP ( 'NONE', ( #2145, #4607, #5123, #1310 ) ) ;
#8540=PRODUCT_DEFINITION_SHAPE ( 'NONE', 'NONE',  #12251 ) ;
#8545=EDGE_CURVE ( 'NONE', #9347, #1577, #8749, .T. ) ;
#8548=CARTESIAN_POINT ( 'NONE',  ( -45.00000000000013500, 30.00000000000000000, 2.000000000000007994 ) ) ;
#8556=CARTESIAN_POINT ( 'NONE',  ( -18.00000000000000355, 29.99999999999998224, 3.000000000000008438 ) ) ;
#8562=CARTESIAN_POINT ( 'NONE',  ( -17.00000000000000000, 30.00000000000000000, 3.000000000000030198 ) ) ;
#8579=DIRECTION ( 'NONE',  ( -1.000000000000000000, -5.916456789157575403E-31, -2.465190328815656418E-32 ) ) ;
#8584=PLANE ( 'NONE',  #5747 ) ;
#8602=ADVANCED_FACE ( 'NONE', ( #7825 ), #11758, .T. ) ;
#8625=AXIS2_PLACEMENT_3D ( 'NONE', #5805, #10950, #17 ) ;
#8648=DIRECTION ( 'NONE',  ( 1.224646799147352714E-16, 1.177425296209236909E-30, 1.000000000000000000 ) ) ;
#8653=UNCERTAINTY_MEASURE_WITH_UNIT (LENGTH_MEASURE( 1.000000000000000082E-05 ), #280, 'distance_accuracy_value', 'NONE');
#8666=VERTEX_POINT ( 'NONE', #9217 ) ;
#8669=VERTEX_POINT ( 'NONE', #3267 ) ;
#8679=CARTESIAN_POINT ( 'NONE',  ( -45.00000000000013500, 30.00000000000000000, 2.000000000000007994 ) ) ;
#8688=FACE_BOUND ( 'NONE', #8932, .T. ) ;
#8690=EDGE_CURVE ( 'NONE', #364, #11848, #703, .T. ) ;
#8731=ORIENTED_EDGE ( 'NONE', *, *, #1114, .F. ) ;
#8743=VECTOR ( 'NONE', #6927, 1000.000000000000000 ) ;
#8746=ORIENTED_EDGE ( 'NONE', *, *, #12415, .F. ) ;
#8749=CIRCLE ( 'NONE', #3223, 3.000000000000005773 ) ;
#8751=AXIS2_PLACEMENT_3D ( 'NONE', #782, #8648, #6533 ) ;
#8753=ORIENTED_EDGE ( 'NONE', *, *, #4877, .F. ) ;
#8771=CYLINDRICAL_SURFACE ( 'NONE', #8625, 2.149999999999999023 ) ;
#8814=VECTOR ( 'NONE', #11987, 1000.000000000000000 ) ;
#8844=FACE_OUTER_BOUND ( 'NONE', #11523, .T. ) ;
#8893=CARTESIAN_POINT ( 'NONE',  ( -18.00000000000001421, -30.00000000000001421, 3.000000000000008438 ) ) ;
#8913=VERTEX_POINT ( 'NONE', #538 ) ;
#8914=PRODUCT_CONTEXT ( 'NONE', #2825, 'mechanical' ) ;
#8927=ORIENTED_EDGE ( 'NONE', *, *, #213, .F. ) ;
#8932=EDGE_LOOP ( 'NONE', ( #12478, #8927 ) ) ;
#8946=DIRECTION ( 'NONE',  ( 1.000000000000000000, 0.000000000000000000, -6.375108774214761023E-14 ) ) ;
#8950=CARTESIAN_POINT ( 'NONE',  ( -17.00000000000000000, 2.632990618166785569E-16, 17.85000000000008313 ) ) ;
#8952=DIRECTION ( 'NONE',  ( 1.577021341797099039E-16, 1.177425296209237084E-30, 1.000000000000000000 ) ) ;
#8953=EDGE_CURVE ( 'NONE', #1577, #8666, #1941, .T. ) ;
#8971=CARTESIAN_POINT ( 'NONE',  ( -17.00000000000000000, 0.000000000000000000, 20.00000000000007461 ) ) ;
#9020=ADVANCED_FACE ( 'NONE', ( #9659 ), #8771, .F. ) ;
#9024=CYLINDRICAL_SURFACE ( 'NONE', #6135, 3.000000000000005773 ) ;
#9026=ORIENTED_EDGE ( 'NONE', *, *, #1708, .T. ) ;
#9032=DIRECTION ( 'NONE',  ( -4.930380657631325535E-31, -1.000000000000000000, -1.177425296209239362E-30 ) ) ;
#9052=COLOUR_RGB ( '', 0.66274510, 0.83137255, 0.94901961) ;
#9057=EDGE_LOOP ( 'NONE', ( #11975, #5276, #822, #5828 ) ) ;
#9078=CYLINDRICAL_SURFACE ( 'NONE', #3546, 1.000000000000001332 ) ;
#9111=EDGE_CURVE ( 'NONE', #7500, #302, #5128, .T. ) ;
#9121=DIRECTION ( 'NONE',  ( -1.000000000000000000, 0.000000000000000000, 1.301042606982602363E-16 ) ) ;
#9173=ADVANCED_FACE ( 'NONE', ( #3252, #11086 ), #7355, .T. ) ;
#9194=CARTESIAN_POINT ( 'NONE',  ( -37.15000000000005542, 2.632990618166571591E-16, 2.431703406787713260E-15 ) ) ;
#9204=APPLICATION_CONTEXT ( 'automotive_design' ) ;
#9217=CARTESIAN_POINT ( 'NONE',  ( -15.00000000000000711, -30.00000000000000000, 25.00000000000007105 ) ) ;
#9229=DIRECTION ( 'NONE',  ( 2.465190328815656418E-32, -1.177425296209236734E-30, -1.000000000000000000 ) ) ;
#9281=PLANE ( 'NONE',  #3015 ) ;
#9310=VERTEX_POINT ( 'NONE', #2592 ) ;
#9347=VERTEX_POINT ( 'NONE', #522 ) ;
#9378=ORIENTED_EDGE ( 'NONE', *, *, #6612, .F. ) ;
#9403=ADVANCED_FACE ( 'NONE', ( #9768 ), #834, .F. ) ;
#9411=CARTESIAN_POINT ( 'NONE',  ( -15.00000000000000000, -19.99999999999998934, 12.00000000000002842 ) ) ;
#9430=DIRECTION ( 'NONE',  ( -1.000000000000000000, -5.916456789157575403E-31, 1.577021341797099039E-16 ) ) ;
#9458=EDGE_CURVE ( 'NONE', #7454, #10609, #1019, .T. ) ;
#9544=ORIENTED_EDGE ( 'NONE', *, *, #3145, .T. ) ;
#9576=AXIS2_PLACEMENT_3D ( 'NONE', #5692, #11438, #4734 ) ;
#9611=VERTEX_POINT ( 'NONE', #10088 ) ;
#9630=CARTESIAN_POINT ( 'NONE',  ( -37.15000000000006253, 2.632990618166587368E-16, 2.000000000000002220 ) ) ;
#9659=FACE_OUTER_BOUND ( 'NONE', #7704, .T. ) ;
#9663=VERTEX_POINT ( 'NONE', #5531 ) ;
#9675=ORIENTED_EDGE ( 'NONE', *, *, #12697, .F. ) ;
#9679=( NAMED_UNIT ( * ) SI_UNIT ( $, .STERADIAN. ) SOLID_ANGLE_UNIT ( ) );
#9701=ADVANCED_BREP_SHAPE_REPRESENTATION ( '', ( #10029, #12422 ), #5765 ) ;
#9703=CARTESIAN_POINT ( 'NONE',  ( -35.00000000000006395, -2.157041537713704155E-29, 2.000000000000002220 ) ) ;
#9709=DIRECTION ( 'NONE',  ( -1.000000000000000000, -5.916456789157576279E-31, 1.224646799147353947E-16 ) ) ;
#9745=VECTOR ( 'NONE', #1402, 1000.000000000000000 ) ;
#9765=DIRECTION ( 'NONE',  ( -1.577021341797098546E-16, -1.177425296209237084E-30, -1.000000000000000000 ) ) ;
#9768=FACE_OUTER_BOUND ( 'NONE', #11708, .T. ) ;
#9769=CIRCLE ( 'NONE', #5480, 2.149999999999999023 ) ;
#9777=ADVANCED_FACE ( 'NONE', ( #11464, #2648, #2635, #2500 ), #3408, .T. ) ;
#9795=EDGE_LOOP ( 'NONE', ( #55, #546, #9026, #4213 ) ) ;
#9914=VECTOR ( 'NONE', #2233, 1000.000000000000000 ) ;
#9926=FACE_OUTER_BOUND ( 'NONE', #2697, .T. ) ;
#9964=ORIENTED_EDGE ( 'NONE', *, *, #8953, .F. ) ;
#9978=DIRECTION ( 'NONE',  ( -1.000000000000000000, -5.916456789157575403E-31, 1.577021341797098793E-16 ) ) ;
#9980=DIRECTION ( 'NONE',  ( -1.000000000000000000, -5.916456789157575403E-31, 1.577021341797098793E-16 ) ) ;
#10007=ORIENTED_EDGE ( 'NONE', *, *, #6653, .T. ) ;
#10014=CARTESIAN_POINT ( 'NONE',  ( -35.00000000000006395, -19.99999999999999645, 2.000000000000006661 ) ) ;
#10026=EDGE_LOOP ( 'NONE', ( #4746, #1146 ) ) ;
#10029=MANIFOLD_SOLID_BREP ( 'M4 Clearance Hole2', #12623 ) ;
#10034=DIRECTION ( 'NONE',  ( 0.000000000000000000, 0.000000000000000000, 1.000000000000000000 ) ) ;
#10051=DIRECTION ( 'NONE',  ( -1.224646799147352714E-16, -1.177425296209236909E-30, -1.000000000000000000 ) ) ;
#10079=CARTESIAN_POINT ( 'NONE',  ( -15.00000000000000000, -19.99999999999998934, 12.00000000000002842 ) ) ;
#10086=ADVANCED_FACE ( 'NONE', ( #9926 ), #1118, .F. ) ;
#10088=CARTESIAN_POINT ( 'NONE',  ( -45.00000000000012079, -19.99999999999999645, 3.443468848353431668E-15 ) ) ;
#10107=SHAPE_REPRESENTATION_RELATIONSHIP ( 'NONE' , 'NONE' ,  #11514, #9701 ) ;
#10116=DIRECTION ( 'NONE',  ( -1.000000000000000000, -5.916456789157575403E-31, 1.224646799147352714E-16 ) ) ;
#10120=ORIENTED_EDGE ( 'NONE', *, *, #3773, .F. ) ;
#10126=ORIENTED_EDGE ( 'NONE', *, *, #5714, .T. ) ;
#10180=VERTEX_POINT ( 'NONE', #472 ) ;
#10186=CYLINDRICAL_SURFACE ( 'NONE', #4876, 10.00000000000002309 ) ;
#10265=AXIS2_PLACEMENT_3D ( 'NONE', #9703, #12635, #10869 ) ;
#10278=CARTESIAN_POINT ( 'NONE',  ( -35.00000000000006395, 30.00000000000000000, 2.000000000000007994 ) ) ;
#10302=ORIENTED_EDGE ( 'NONE', *, *, #5301, .T. ) ;
#10305=LINE ( 'NONE', #1561, #6112 ) ;
#10315=ADVANCED_FACE ( 'NONE', ( #6538 ), #8584, .T. ) ;
#10319=CYLINDRICAL_SURFACE ( 'NONE', #2129, 2.149999999999999023 ) ;
#10320=VECTOR ( 'NONE', #3795, 1000.000000000000000 ) ;
#10365=CARTESIAN_POINT ( 'NONE',  ( -17.00000000000000000, 0.000000000000000000, 20.00000000000007461 ) ) ;
#10406=LINE ( 'NONE', #8291, #799 ) ;
#10412=EDGE_CURVE ( 'NONE', #4937, #10180, #10687, .T. ) ;
#10453=ORIENTED_EDGE ( 'NONE', *, *, #7577, .T. ) ;
#10517=ORIENTED_EDGE ( 'NONE', *, *, #5923, .T. ) ;
#10523=ORIENTED_EDGE ( 'NONE', *, *, #11922, .F. ) ;
#10535=DIRECTION ( 'NONE',  ( -2.465190328815656418E-32, 1.177425296209236734E-30, 1.000000000000000000 ) ) ;
#10542=AXIS2_PLACEMENT_3D ( 'NONE', #6133, #9978, #12068 ) ;
#10546=FACE_OUTER_BOUND ( 'NONE', #11272, .T. ) ;
#10559=DIRECTION ( 'NONE',  ( 0.000000000000000000, 1.177425296209237785E-30, 1.000000000000000000 ) ) ;
#10563=CARTESIAN_POINT ( 'NONE',  ( -18.00000000000002842, 30.00000000000000000, 4.336808689942017736E-16 ) ) ;
#10574=EDGE_CURVE ( 'NONE', #8669, #4937, #4706, .T. ) ;
#10584=DIRECTION ( 'NONE',  ( -1.000000000000000000, -5.916456789157576279E-31, 1.224646799147353947E-16 ) ) ;
#10609=VERTEX_POINT ( 'NONE', #11602 ) ;
#10633=LINE ( 'NONE', #6784, #7117 ) ;
#10645=DIRECTION ( 'NONE',  ( 0.000000000000000000, 1.177425296209236909E-30, 1.000000000000000000 ) ) ;
#10660=CARTESIAN_POINT ( 'NONE',  ( -17.00000000000002842, 19.99999999999998579, 9.850000000000047606 ) ) ;
#10687=CIRCLE ( 'NONE', #5963, 1.000000000000000888 ) ;
#10695=MECHANICAL_DESIGN_GEOMETRIC_PRESENTATION_REPRESENTATION('',(#3519),#11123);
#10714=EDGE_CURVE ( 'NONE', #7082, #8913, #12749, .T. ) ;
#10774=SURFACE_STYLE_FILL_AREA ( #7052 ) ;
#10832=DIRECTION ( 'NONE',  ( -2.465190328815656418E-32, 1.177425296209236909E-30, 1.000000000000000000 ) ) ;
#10838=CARTESIAN_POINT ( 'NONE',  ( -45.00000000000012079, -19.99999999999999645, 2.000000000000007994 ) ) ;
#10869=DIRECTION ( 'NONE',  ( 1.000000000000000000, 5.916456789157576279E-31, 0.000000000000000000 ) ) ;
#10913=CARTESIAN_POINT ( 'NONE',  ( -18.00000000000002842, -30.00000000000000000, 2.000000000000004441 ) ) ;
#10950=DIRECTION ( 'NONE',  ( -1.000000000000000000, -5.916456789157575403E-31, 1.577021341797098793E-16 ) ) ;
#10955=( LENGTH_UNIT ( ) NAMED_UNIT ( * ) SI_UNIT ( .MILLI., .METRE. ) );
#10966=EDGE_CURVE ( 'NONE', #11848, #4250, #681, .T. ) ;
#10980=AXIS2_PLACEMENT_3D ( 'NONE', #279, #12146, #471 ) ;
#11023=DIRECTION ( 'NONE',  ( -1.000000000000000000, -5.916456789157575403E-31, -2.465190328815656418E-32 ) ) ;
#11028=ORIENTED_EDGE ( 'NONE', *, *, #8545, .F. ) ;
#11077=EDGE_CURVE ( 'NONE', #12092, #3334, #1962, .T. ) ;
#11086=FACE_OUTER_BOUND ( 'NONE', #6809, .T. ) ;
#11091=PRESENTATION_STYLE_ASSIGNMENT (( #6812 ) ) ;
#11123=( GEOMETRIC_REPRESENTATION_CONTEXT ( 3 ) GLOBAL_UNCERTAINTY_ASSIGNED_CONTEXT ( ( #4788 ) ) GLOBAL_UNIT_ASSIGNED_CONTEXT ( ( #10955, #2143, #9679 ) ) REPRESENTATION_CONTEXT ( 'NONE', 'WORKASPACE' ) );
#11157=AXIS2_PLACEMENT_3D ( 'NONE', #8556, #3734, #5535 ) ;
#11162=CYLINDRICAL_SURFACE ( 'NONE', #4262, 2.149999999999999023 ) ;
#11187=EDGE_LOOP ( 'NONE', ( #8408, #565, #2912, #10517 ) ) ;
#11203=PRODUCT_DEFINITION_CONTEXT ( 'detailed design', #9204, 'design' ) ;
#11229=LINE ( 'NONE', #4331, #12225 ) ;
#11240=ORIENTED_EDGE ( 'NONE', *, *, #3183, .T. ) ;
#11249=AXIS2_PLACEMENT_3D ( 'NONE', #548, #734, #2494 ) ;
#11253=ORIENTED_EDGE ( 'NONE', *, *, #12415, .T. ) ;
#11267=LINE ( 'NONE', #10278, #11418 ) ;
#11272=EDGE_LOOP ( 'NONE', ( #8746, #6560, #12545, #11696, #10126, #1071, #5061, #5713 ) ) ;
#11279=CARTESIAN_POINT ( 'NONE',  ( -18.00000000000002842, 30.00000000000000000, 1.369224906555730040E-16 ) ) ;
#11295=AXIS2_PLACEMENT_3D ( 'NONE', #263, #6062, #1166 ) ;
#11382=ORIENTED_EDGE ( 'NONE', *, *, #6239, .F. ) ;
#11397=DIRECTION ( 'NONE',  ( -4.930380657631325535E-31, -1.000000000000000000, -1.177425296209239362E-30 ) ) ;
#11405=CARTESIAN_POINT ( 'NONE',  ( -18.00000000000002842, 30.00000000000000000, 1.369224906555730040E-16 ) ) ;
#11418=VECTOR ( 'NONE', #5397, 1000.000000000000000 ) ;
#11438=DIRECTION ( 'NONE',  ( -2.465190328815656418E-32, 1.177425296209236734E-30, 1.000000000000000000 ) ) ;
#11464=FACE_BOUND ( 'NONE', #10026, .T. ) ;
#11494=UNCERTAINTY_MEASURE_WITH_UNIT (LENGTH_MEASURE( 1.000000000000000082E-05 ), #1779, 'distance_accuracy_value', 'NONE');
#11498=VERTEX_POINT ( 'NONE', #1693 ) ;
#11514=SHAPE_REPRESENTATION ( 'cover 2', ( #12422 ), #5765 ) ;
#11518=CARTESIAN_POINT ( 'NONE',  ( -37.15000000000005542, 2.632990618166567153E-16, 2.000000000000003553 ) ) ;
#11523=EDGE_LOOP ( 'NONE', ( #7118, #5583, #6569, #5423 ) ) ;
#11530=CIRCLE ( 'NONE', #5141, 2.149999999999999023 ) ;
#11550=CARTESIAN_POINT ( 'NONE',  ( -35.00000000000006395, -2.157041537713704155E-29, 2.168404344971033323E-15 ) ) ;
#11559=DIRECTION ( 'NONE',  ( 5.916456789157575403E-31, -1.000000000000000000, -1.177425296209239362E-30 ) ) ;
#11570=ORIENTED_EDGE ( 'NONE', *, *, #2597, .F. ) ;
#11585=ORIENTED_EDGE ( 'NONE', *, *, #6529, .F. ) ;
#11587=CARTESIAN_POINT ( 'NONE',  ( -15.00000000000000000, -20.00000000000000000, 9.850000000000033396 ) ) ;
#11602=CARTESIAN_POINT ( 'NONE',  ( -17.00000000000002842, -20.00000000000000000, 14.15000000000003055 ) ) ;
#11642=CARTESIAN_POINT ( 'NONE',  ( -17.00000000000002842, -20.00000000000000000, 14.15000000000003588 ) ) ;
#11665=VERTEX_POINT ( 'NONE', #80 ) ;
#11696=ORIENTED_EDGE ( 'NONE', *, *, #11983, .T. ) ;
#11699=DIRECTION ( 'NONE',  ( -1.000000000000000000, -5.916456789157575403E-31, 1.577021341797099039E-16 ) ) ;
#11701=ORIENTED_EDGE ( 'NONE', *, *, #1864, .F. ) ;
#11708=EDGE_LOOP ( 'NONE', ( #582, #2894, #2262, #11570 ) ) ;
#11758=CYLINDRICAL_SURFACE ( 'NONE', #1932, 10.00000000000002309 ) ;
#11760=FILL_AREA_STYLE_COLOUR ( '', #9052 ) ;
#11781=CIRCLE ( 'NONE', #2949, 1.000000000000000888 ) ;
#11792=EDGE_CURVE ( 'NONE', #509, #47, #8046, .T. ) ;
#11806=LINE ( 'NONE', #7164, #4469 ) ;
#11816=CARTESIAN_POINT ( 'NONE',  ( -14.99999999999999289, 30.00000000000000000, 25.00000000000007105 ) ) ;
#11845=ORIENTED_EDGE ( 'NONE', *, *, #5959, .F. ) ;
#11848=VERTEX_POINT ( 'NONE', #2595 ) ;
#11854=DIRECTION ( 'NONE',  ( 0.000000000000000000, 0.000000000000000000, 1.000000000000000000 ) ) ;
#11901=CIRCLE ( 'NONE', #7407, 2.149999999999999023 ) ;
#11921=CARTESIAN_POINT ( 'NONE',  ( -45.00000000000001421, 19.99999999999999645, 2.000000000000007994 ) ) ;
#11922=EDGE_CURVE ( 'NONE', #4963, #8313, #5798, .T. ) ;
#11923=CARTESIAN_POINT ( 'NONE',  ( -15.00000000000000000, 30.00000000000000000, 3.000000000000029754 ) ) ;
#11975=ORIENTED_EDGE ( 'NONE', *, *, #1114, .T. ) ;
#11983=EDGE_CURVE ( 'NONE', #8669, #12227, #11781, .T. ) ;
#11987=DIRECTION ( 'NONE',  ( 1.577021341797099039E-16, 1.177425296209237084E-30, 1.000000000000000000 ) ) ;
#11996=DIRECTION ( 'NONE',  ( -1.224646799147352714E-16, -1.177425296209236909E-30, -1.000000000000000000 ) ) ;
#11999=VECTOR ( 'NONE', #240, 1000.000000000000000 ) ;
#12068=DIRECTION ( 'NONE',  ( 0.000000000000000000, 0.000000000000000000, 1.000000000000000000 ) ) ;
#12092=VERTEX_POINT ( 'NONE', #11921 ) ;
#12124=VECTOR ( 'NONE', #7703, 1000.000000000000000 ) ;
#12136=VERTEX_POINT ( 'NONE', #5404 ) ;
#12146=DIRECTION ( 'NONE',  ( -4.930380657631325535E-31, -1.000000000000000000, -1.177425296209239362E-30 ) ) ;
#12165=DIRECTION ( 'NONE',  ( 1.000000000000000000, 5.916456789157575403E-31, -1.577021341797098546E-16 ) ) ;
#12219=CARTESIAN_POINT ( 'NONE',  ( -35.00000000000006395, -2.157041537713704155E-29, 2.000000000000002220 ) ) ;
#12225=VECTOR ( 'NONE', #8260, 1000.000000000000000 ) ;
#12227=VERTEX_POINT ( 'NONE', #4312 ) ;
#12248=DIRECTION ( 'NONE',  ( -1.224646799147352714E-16, -1.177425296209236909E-30, -1.000000000000000000 ) ) ;
#12250=EDGE_CURVE ( 'NONE', #11665, #8458, #8105, .T. ) ;
#12251=PRODUCT_DEFINITION ( 'UNKNOWN', '', #2845, #11203 ) ;
#12256=ORIENTED_EDGE ( 'NONE', *, *, #12250, .T. ) ;
#12277=ORIENTED_EDGE ( 'NONE', *, *, #9458, .F. ) ;
#12284=ADVANCED_FACE ( 'NONE', ( #10546 ), #2583, .F. ) ;
#12309=EDGE_LOOP ( 'NONE', ( #10120, #3143, #4231, #6018 ) ) ;
#12344=DIRECTION ( 'NONE',  ( -1.000000000000000000, -5.916456789157575403E-31, 1.577021341797098793E-16 ) ) ;
#12376=ORIENTED_EDGE ( 'NONE', *, *, #10714, .F. ) ;
#12378=LINE ( 'NONE', #11405, #61 ) ;
#12398=EDGE_CURVE ( 'NONE', #8313, #1734, #5719, .T. ) ;
#12415=EDGE_CURVE ( 'NONE', #12136, #364, #12378, .T. ) ;
#12418=VECTOR ( 'NONE', #4282, 1000.000000000000000 ) ;
#12422=AXIS2_PLACEMENT_3D ( 'NONE', #5707, #7392, #6428 ) ;
#12426=LINE ( 'NONE', #7457, #3283 ) ;
#12466=CIRCLE ( 'NONE', #8751, 10.00000000000002309 ) ;
#12474=CARTESIAN_POINT ( 'NONE',  ( -15.00000000000000000, 2.632990618166788035E-16, 17.85000000000007958 ) ) ;
#12478=ORIENTED_EDGE ( 'NONE', *, *, #5431, .F. ) ;
#12482=( NAMED_UNIT ( * ) PLANE_ANGLE_UNIT ( ) SI_UNIT ( $, .RADIAN. ) );
#12517=CARTESIAN_POINT ( 'NONE',  ( -15.00000000000003375, 19.99999999999998579, 14.15000000000002167 ) ) ;
#12520=DIRECTION ( 'NONE',  ( -1.224646799147352714E-16, -1.177425296209236909E-30, -1.000000000000000000 ) ) ;
#12522=CIRCLE ( 'NONE', #5750, 2.149999999999999023 ) ;
#12545=ORIENTED_EDGE ( 'NONE', *, *, #6529, .T. ) ;
#12578=CARTESIAN_POINT ( 'NONE',  ( -18.00000000000001421, 29.99999999999999289, 2.000000000000004885 ) ) ;
#12623=CLOSED_SHELL ( 'NONE', ( #9020, #10086, #3362, #9403, #766, #1296, #9777, #1318, #9173, #4319, #7340, #606, #12284, #10315, #8602, #5809, #3407, #6086, #4740, #7242 ) ) ;
#12624=EDGE_LOOP ( 'NONE', ( #5913, #12277 ) ) ;
#12635=DIRECTION ( 'NONE',  ( -2.465190328815656418E-32, 1.177425296209236734E-30, 1.000000000000000000 ) ) ;
#12637=DIRECTION ( 'NONE',  ( 1.000000000000000000, 5.916456789157575403E-31, -1.577021341797098793E-16 ) ) ;
#12662=CARTESIAN_POINT ( 'NONE',  ( -35.00000000000006395, -30.00000000000000000, 3.000000000000008438 ) ) ;
#12692=VECTOR ( 'NONE', #6430, 1000.000000000000000 ) ;
#12697=EDGE_CURVE ( 'NONE', #364, #9347, #6102, .T. ) ;
#12715=EDGE_CURVE ( 'NONE', #7976, #9310, #4796, .T. ) ;
#12728=LINE ( 'NONE', #6803, #8743 ) ;
#12749=CIRCLE ( 'NONE', #1639, 2.149999999999999023 ) ;
ENDSEC;
END-ISO-10303-21;
